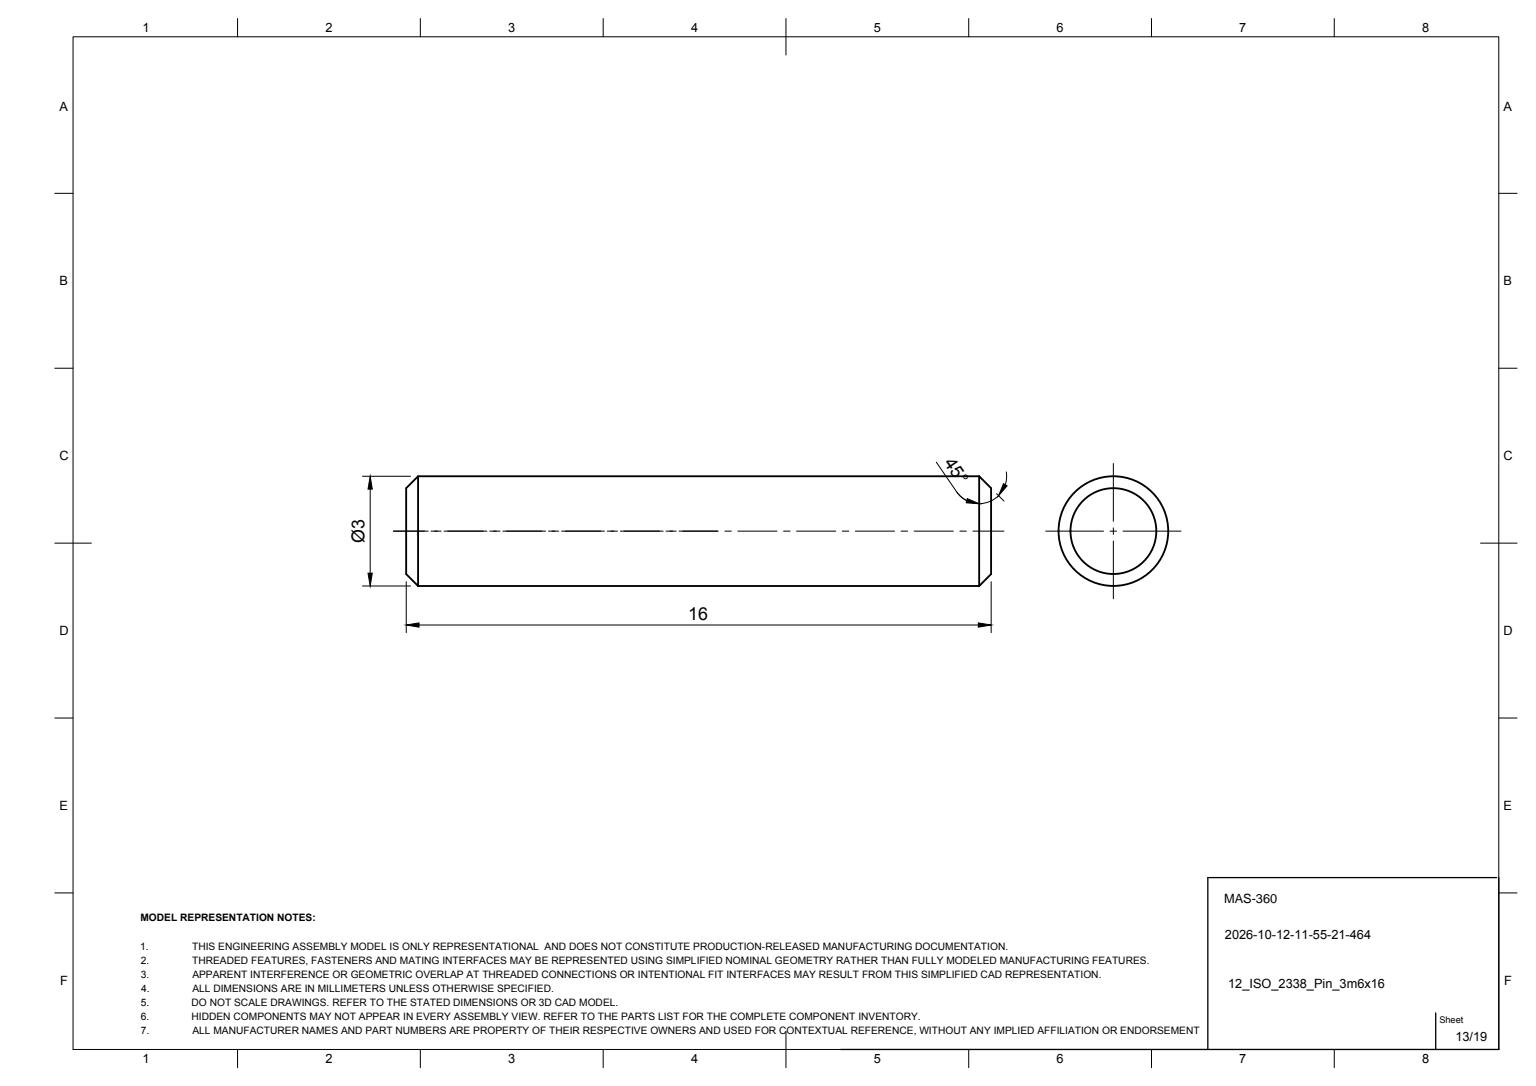
ISO-10303-21;
HEADER;
/* Generated by software containing ST-Developer
 * from STEP Tools, Inc. (www.steptools.com) 
 */

FILE_DESCRIPTION(
/* description */ (''),
/* implementation_level */ '2;1');

FILE_NAME(
/* name */ '12_ISO_2338_Pin_3m6x16.step',
/* time_stamp */ '2026-11-04T18:53:29-08:00',
/* author */ (''),
/* organization */ (''),
/* preprocessor_version */ 'ST-DEVELOPER v20.2',
/* originating_system */ 'Autodesk Translation Framework v15.17.0.0',
/* authorisation */ '');

FILE_SCHEMA (('AUTOMOTIVE_DESIGN { 1 0 10303 214 3 1 1 }'));
ENDSEC;

DATA;
#10=MECHANICAL_DESIGN_GEOMETRIC_PRESENTATION_REPRESENTATION('',(#1339),#100031);
#239=CONICAL_SURFACE('',#22418,1.3368,0.785398163397446);
#240=CONICAL_SURFACE('',#22423,1.3368,0.785398163397446);
#1148=CIRCLE('',#22419,1.5);
#1149=CIRCLE('',#22420,1.1736);
#1150=CIRCLE('',#22422,1.5);
#1151=CIRCLE('',#22424,1.1736);
#1303=SHAPE_REPRESENTATION_RELATIONSHIP('SRR','None',#100113,#1321);
#1321=ADVANCED_BREP_SHAPE_REPRESENTATION('',(#1357),#100025);
#1339=STYLED_ITEM('',(#100203),#1357);
#1357=MANIFOLD_SOLID_BREP('Body1',#20129);
#1677=PLANE('',#22425);
#1678=PLANE('',#22426);
#3245=LINE('',#99832,#4532);
#3246=LINE('',#99837,#4533);
#3247=LINE('',#99840,#4534);
#4532=VECTOR('',#27962,1.3368);
#4533=VECTOR('',#27969,1.5);
#4534=VECTOR('',#27972,1.3368);
#5015=CYLINDRICAL_SURFACE('',#22421,1.5);
#6142=FACE_OUTER_BOUND('',#7409,.T.);
#6143=FACE_OUTER_BOUND('',#7410,.T.);
#6144=FACE_OUTER_BOUND('',#7411,.T.);
#6145=FACE_OUTER_BOUND('',#7412,.T.);
#6146=FACE_OUTER_BOUND('',#7413,.T.);
#7409=EDGE_LOOP('',(#18735,#18736,#18737,#18738));
#7410=EDGE_LOOP('',(#18739,#18740,#18741,#18742));
#7411=EDGE_LOOP('',(#18743,#18744,#18745,#18746));
#7412=EDGE_LOOP('',(#18747));
#7413=EDGE_LOOP('',(#18748));
#9889=VERTEX_POINT('',#99829);
#9890=VERTEX_POINT('',#99831);
#9891=VERTEX_POINT('',#99835);
#9892=VERTEX_POINT('',#99839);
#12842=EDGE_CURVE('',#9889,#9889,#1148,.T.);
#12843=EDGE_CURVE('',#9889,#9890,#3245,.T.);
#12844=EDGE_CURVE('',#9890,#9890,#1149,.T.);
#12845=EDGE_CURVE('',#9891,#9891,#1150,.T.);
#12846=EDGE_CURVE('',#9891,#9889,#3246,.T.);
#12847=EDGE_CURVE('',#9891,#9892,#3247,.T.);
#12848=EDGE_CURVE('',#9892,#9892,#1151,.T.);
#18735=ORIENTED_EDGE('',*,*,#12842,.F.);
#18736=ORIENTED_EDGE('',*,*,#12843,.T.);
#18737=ORIENTED_EDGE('',*,*,#12844,.T.);
#18738=ORIENTED_EDGE('',*,*,#12843,.F.);
#18739=ORIENTED_EDGE('',*,*,#12845,.F.);
#18740=ORIENTED_EDGE('',*,*,#12846,.T.);
#18741=ORIENTED_EDGE('',*,*,#12842,.T.);
#18742=ORIENTED_EDGE('',*,*,#12846,.F.);
#18743=ORIENTED_EDGE('',*,*,#12845,.T.);
#18744=ORIENTED_EDGE('',*,*,#12847,.T.);
#18745=ORIENTED_EDGE('',*,*,#12848,.F.);
#18746=ORIENTED_EDGE('',*,*,#12847,.F.);
#18747=ORIENTED_EDGE('',*,*,#12848,.T.);
#18748=ORIENTED_EDGE('',*,*,#12844,.F.);
#20076=ADVANCED_FACE('',(#6142),#239,.T.);
#20077=ADVANCED_FACE('',(#6143),#5015,.T.);
#20078=ADVANCED_FACE('',(#6144),#240,.T.);
#20079=ADVANCED_FACE('',(#6145),#1677,.T.);
#20080=ADVANCED_FACE('',(#6146),#1678,.T.);
#20129=CLOSED_SHELL('',(#20076,#20077,#20078,#20079,#20080));
#22417=AXIS2_PLACEMENT_3D('',#99827,#27956,#27957);
#22418=AXIS2_PLACEMENT_3D('',#99828,#27958,#27959);
#22419=AXIS2_PLACEMENT_3D('',#99830,#27960,#27961);
#22420=AXIS2_PLACEMENT_3D('',#99833,#27963,#27964);
#22421=AXIS2_PLACEMENT_3D('',#99834,#27965,#27966);
#22422=AXIS2_PLACEMENT_3D('',#99836,#27967,#27968);
#22423=AXIS2_PLACEMENT_3D('',#99838,#27970,#27971);
#22424=AXIS2_PLACEMENT_3D('',#99841,#27973,#27974);
#22425=AXIS2_PLACEMENT_3D('',#99842,#27975,#27976);
#22426=AXIS2_PLACEMENT_3D('',#99843,#27977,#27978);
#27956=DIRECTION('axis',(0.,0.,1.));
#27957=DIRECTION('refdir',(1.,0.,0.));
#27958=DIRECTION('center_axis',(1.,0.,0.));
#27959=DIRECTION('ref_axis',(0.,1.,0.));
#27960=DIRECTION('center_axis',(1.,0.,0.));
#27961=DIRECTION('ref_axis',(0.,0.,-1.));
#27962=DIRECTION('',(-0.707106781186549,0.707106781186546,8.65956056235491E-17));
#27963=DIRECTION('center_axis',(1.,0.,0.));
#27964=DIRECTION('ref_axis',(0.,0.,-1.));
#27965=DIRECTION('center_axis',(1.,0.,0.));
#27966=DIRECTION('ref_axis',(0.,1.,0.));
#27967=DIRECTION('center_axis',(1.,0.,0.));
#27968=DIRECTION('ref_axis',(0.,0.,-1.));
#27969=DIRECTION('',(-1.,0.,0.));
#27970=DIRECTION('center_axis',(-1.,0.,0.));
#27971=DIRECTION('ref_axis',(0.,1.,0.));
#27972=DIRECTION('',(0.707106781186549,0.707106781186546,-8.65956056235491E-17));
#27973=DIRECTION('center_axis',(1.,0.,0.));
#27974=DIRECTION('ref_axis',(0.,0.,-1.));
#27975=DIRECTION('center_axis',(1.,0.,0.));
#27976=DIRECTION('ref_axis',(0.,0.,-1.));
#27977=DIRECTION('center_axis',(-1.,0.,0.));
#27978=DIRECTION('ref_axis',(0.,0.,1.));
#99827=CARTESIAN_POINT('',(0.,0.,0.));
#99828=CARTESIAN_POINT('Origin',(-7.8368,0.,0.));
#99829=CARTESIAN_POINT('',(-7.6736,-1.5,-1.83697019872103E-16));
#99830=CARTESIAN_POINT('Origin',(-7.6736,0.,0.));
#99831=CARTESIAN_POINT('',(-8.,-1.1736,-1.43724548347933E-16));
#99832=CARTESIAN_POINT('',(-7.8368,-1.3368,-1.63710784110018E-16));
#99833=CARTESIAN_POINT('Origin',(-8.,0.,0.));
#99834=CARTESIAN_POINT('Origin',(0.,0.,0.));
#99835=CARTESIAN_POINT('',(7.6736,-1.5,-1.83697019872103E-16));
#99836=CARTESIAN_POINT('Origin',(7.6736,0.,0.));
#99837=CARTESIAN_POINT('',(0.,-1.5,-1.83697019872103E-16));
#99838=CARTESIAN_POINT('Origin',(7.8368,0.,0.));
#99839=CARTESIAN_POINT('',(8.,-1.1736,-1.43724548347933E-16));
#99840=CARTESIAN_POINT('',(7.8368,-1.3368,1.63710784110018E-16));
#99841=CARTESIAN_POINT('Origin',(8.,0.,0.));
#99842=CARTESIAN_POINT('Origin',(8.,0.,0.));
#99843=CARTESIAN_POINT('Origin',(-8.,1.1736,0.));
#100005=UNCERTAINTY_MEASURE_WITH_UNIT(LENGTH_MEASURE(0.01),#100032,
'DISTANCE_ACCURACY_VALUE',
'Maximum model space distance between geometric entities at asserted c
onnectivities');
#100011=UNCERTAINTY_MEASURE_WITH_UNIT(LENGTH_MEASURE(0.01),#100032,
'DISTANCE_ACCURACY_VALUE',
'Maximum model space distance between geometric entities at asserted c
onnectivities');
#100025=(
GEOMETRIC_REPRESENTATION_CONTEXT(3)
GLOBAL_UNCERTAINTY_ASSIGNED_CONTEXT((#100005))
GLOBAL_UNIT_ASSIGNED_CONTEXT((#100032,#100034,#100035))
REPRESENTATION_CONTEXT('','3D')
);
#100031=(
GEOMETRIC_REPRESENTATION_CONTEXT(3)
GLOBAL_UNCERTAINTY_ASSIGNED_CONTEXT((#100011))
GLOBAL_UNIT_ASSIGNED_CONTEXT((#100032,#100034,#100035))
REPRESENTATION_CONTEXT('','3D')
);
#100032=(
LENGTH_UNIT()
NAMED_UNIT(*)
SI_UNIT(.MILLI.,.METRE.)
);
#100034=(
NAMED_UNIT(*)
PLANE_ANGLE_UNIT()
SI_UNIT($,.RADIAN.)
);
#100035=(
NAMED_UNIT(*)
SI_UNIT($,.STERADIAN.)
SOLID_ANGLE_UNIT()
);
#100049=SHAPE_DEFINITION_REPRESENTATION(#100068,#100113);
#100068=PRODUCT_DEFINITION_SHAPE('',$,#100133);
#100113=SHAPE_REPRESENTATION('',(#22417),#100025);
#100119=PRODUCT_DEFINITION_CONTEXT('part definition',#100178,'design');
#100133=PRODUCT_DEFINITION('2026-10-12-11-55-21-464',
'12_ISO_2338_Pin_3m6x16',#100152,#100119);
#100152=PRODUCT_DEFINITION_FORMATION('',$,#100193);
#100178=APPLICATION_CONTEXT(
'Core Data for Automotive Mechanical Design Process');
#100179=PRODUCT_CONTEXT('part definition',#100178,'mechanical');
#100193=PRODUCT('2026-10-12-11-55-21-464','12_ISO_2338_Pin_3m6x16',$,(#100179));
#100203=PRESENTATION_STYLE_ASSIGNMENT((#100209));
#100209=SURFACE_STYLE_USAGE(.BOTH.,#100215);
#100215=SURFACE_SIDE_STYLE('',(#100221));
#100221=SURFACE_STYLE_FILL_AREA(#100227);
#100227=FILL_AREA_STYLE('Opaque(122,133,145)',(#100233));
#100233=FILL_AREA_STYLE_COLOUR('Opaque(122,133,145)',#100239);
#100239=COLOUR_RGB('Opaque(122,133,145)',0.47843137254902,0.52156862745098,
0.568627450980392);
ENDSEC;
END-ISO-10303-21;
